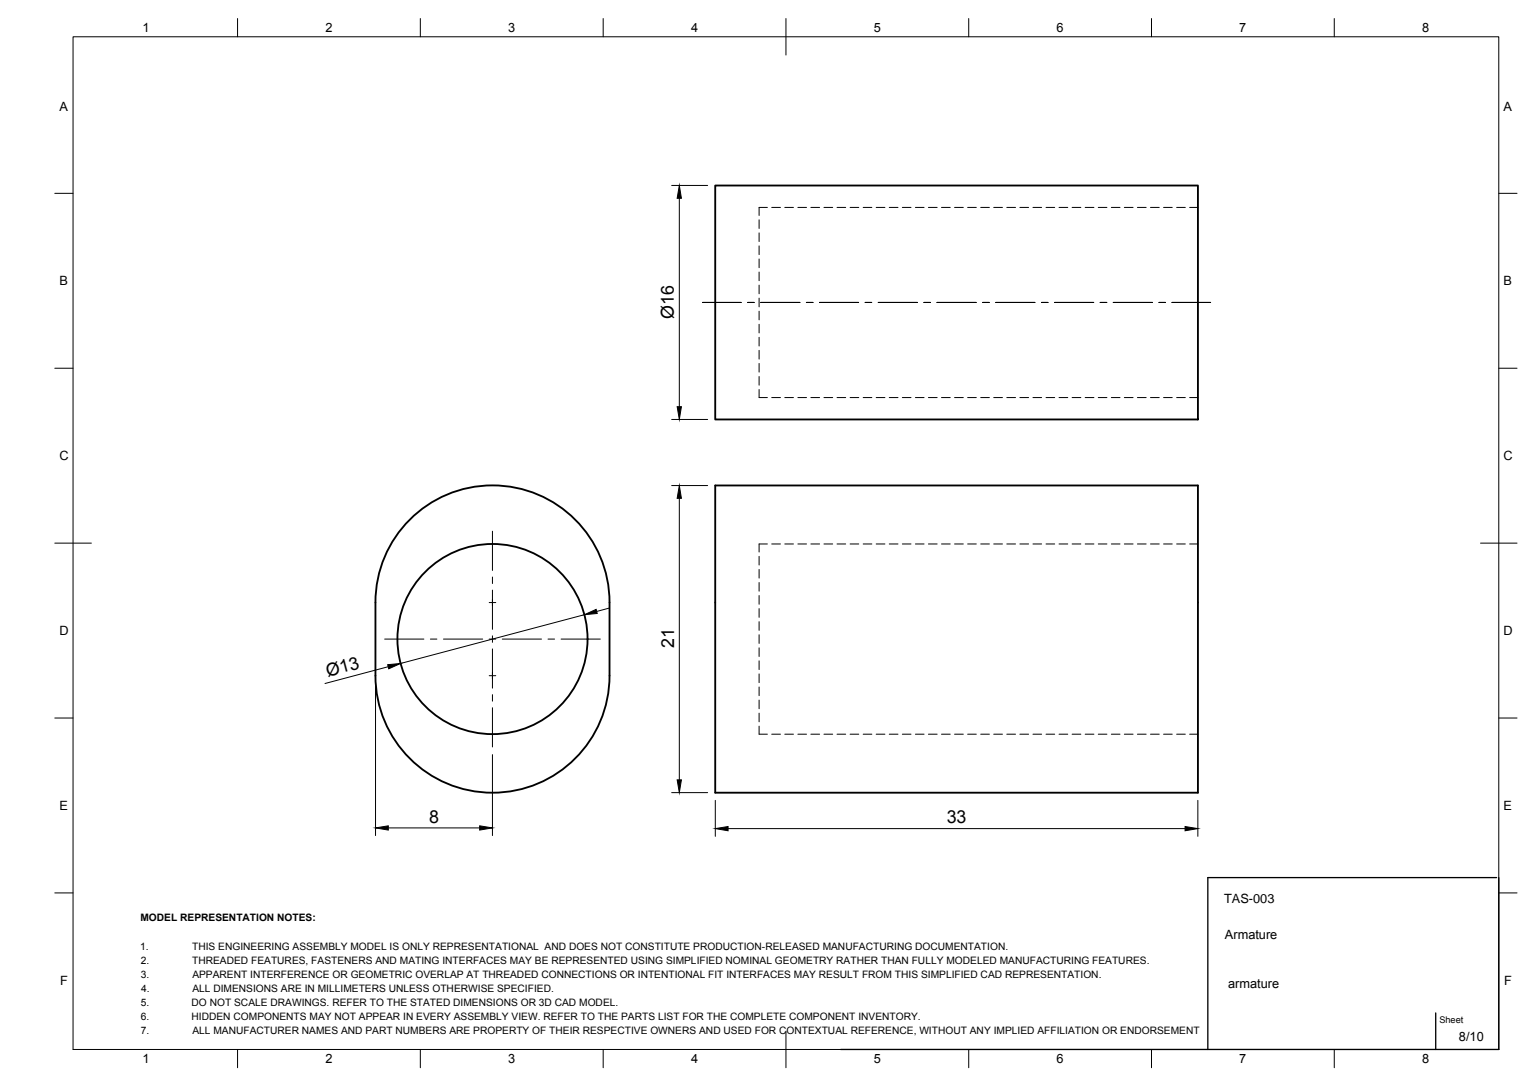
ISO-10303-21;
HEADER;
/* Generated by software containing ST-Developer
 * from STEP Tools, Inc. (www.steptools.com) 
 */

FILE_DESCRIPTION(
/* description */ ('STEP AP214'),
/* implementation_level */ '2;1');

FILE_NAME(
/* name */ 'armature.step',
/* time_stamp */ '2026-11-04T19:43:37-08:00',
/* author */ (''),
/* organization */ (''),
/* preprocessor_version */ 'ST-DEVELOPER v20.2',
/* originating_system */ 'Autodesk Translation Framework v15.17.0.0',
/* authorisation */ '');

FILE_SCHEMA (('AUTOMOTIVE_DESIGN { 1 0 10303 214 3 1 1 }'));
ENDSEC;

DATA;
#10=MECHANICAL_DESIGN_GEOMETRIC_PRESENTATION_REPRESENTATION('',(#120),#7627);
#102=SHAPE_REPRESENTATION_RELATIONSHIP('SRR','None',#7670,#111);
#111=ADVANCED_BREP_SHAPE_REPRESENTATION('',(#141),#7623);
#120=STYLED_ITEM('',(#7723),#141);
#141=MANIFOLD_SOLID_BREP('Body1',#2418);
#178=FACE_BOUND('',#536,.T.);
#217=PLANE('',#2637);
#218=PLANE('',#2641);
#219=PLANE('',#2642);
#220=PLANE('',#2643);
#221=PLANE('',#2644);
#273=CYLINDRICAL_SURFACE('',#2631,6.5);
#274=CYLINDRICAL_SURFACE('',#2634,8.);
#275=CYLINDRICAL_SURFACE('',#2639,8.);
#358=FACE_OUTER_BOUND('',#533,.T.);
#359=FACE_OUTER_BOUND('',#534,.T.);
#360=FACE_OUTER_BOUND('',#535,.T.);
#361=FACE_OUTER_BOUND('',#537,.T.);
#362=FACE_OUTER_BOUND('',#538,.T.);
#363=FACE_OUTER_BOUND('',#539,.T.);
#364=FACE_OUTER_BOUND('',#540,.T.);
#365=FACE_OUTER_BOUND('',#541,.T.);
#533=EDGE_LOOP('',(#1819,#1820,#1821,#1822));
#534=EDGE_LOOP('',(#1823,#1824,#1825,#1826));
#535=EDGE_LOOP('',(#1827,#1828,#1829,#1830));
#536=EDGE_LOOP('',(#1831));
#537=EDGE_LOOP('',(#1832,#1833,#1834,#1835));
#538=EDGE_LOOP('',(#1836,#1837,#1838,#1839));
#539=EDGE_LOOP('',(#1840,#1841,#1842,#1843));
#540=EDGE_LOOP('',(#1844));
#541=EDGE_LOOP('',(#1845,#1846,#1847,#1848));
#689=CIRCLE('',#2632,6.5);
#690=CIRCLE('',#2633,6.5);
#691=CIRCLE('',#2635,8.);
#692=CIRCLE('',#2636,8.);
#693=CIRCLE('',#2638,8.);
#694=CIRCLE('',#2640,8.);
#856=LINE('',#7150,#1012);
#857=LINE('',#7157,#1013);
#858=LINE('',#7160,#1014);
#859=LINE('',#7165,#1015);
#860=LINE('',#7166,#1016);
#861=LINE('',#7169,#1017);
#862=LINE('',#7172,#1018);
#863=LINE('',#7174,#1019);
#864=LINE('',#7176,#1020);
#1012=VECTOR('',#3115,6.5);
#1013=VECTOR('',#3122,1000.);
#1014=VECTOR('',#3125,1000.);
#1015=VECTOR('',#3130,1000.);
#1016=VECTOR('',#3131,1000.);
#1017=VECTOR('',#3134,1000.);
#1018=VECTOR('',#3137,1000.);
#1019=VECTOR('',#3140,1000.);
#1020=VECTOR('',#3143,1000.);
#1181=VERTEX_POINT('',#7147);
#1182=VERTEX_POINT('',#7149);
#1183=VERTEX_POINT('',#7153);
#1184=VERTEX_POINT('',#7154);
#1185=VERTEX_POINT('',#7156);
#1186=VERTEX_POINT('',#7158);
#1187=VERTEX_POINT('',#7162);
#1188=VERTEX_POINT('',#7163);
#1189=VERTEX_POINT('',#7168);
#1190=VERTEX_POINT('',#7170);
#1404=EDGE_CURVE('',#1181,#1181,#689,.T.);
#1405=EDGE_CURVE('',#1181,#1182,#856,.T.);
#1406=EDGE_CURVE('',#1182,#1182,#690,.T.);
#1407=EDGE_CURVE('',#1183,#1184,#691,.T.);
#1408=EDGE_CURVE('',#1183,#1185,#857,.T.);
#1409=EDGE_CURVE('',#1185,#1186,#692,.T.);
#1410=EDGE_CURVE('',#1184,#1186,#858,.T.);
#1411=EDGE_CURVE('',#1187,#1188,#693,.T.);
#1412=EDGE_CURVE('',#1186,#1187,#859,.T.);
#1413=EDGE_CURVE('',#1188,#1185,#860,.T.);
#1414=EDGE_CURVE('',#1189,#1188,#861,.T.);
#1415=EDGE_CURVE('',#1190,#1189,#694,.T.);
#1416=EDGE_CURVE('',#1190,#1187,#862,.T.);
#1417=EDGE_CURVE('',#1189,#1183,#863,.T.);
#1418=EDGE_CURVE('',#1184,#1190,#864,.T.);
#1819=ORIENTED_EDGE('',*,*,#1404,.T.);
#1820=ORIENTED_EDGE('',*,*,#1405,.T.);
#1821=ORIENTED_EDGE('',*,*,#1406,.F.);
#1822=ORIENTED_EDGE('',*,*,#1405,.F.);
#1823=ORIENTED_EDGE('',*,*,#1407,.F.);
#1824=ORIENTED_EDGE('',*,*,#1408,.T.);
#1825=ORIENTED_EDGE('',*,*,#1409,.T.);
#1826=ORIENTED_EDGE('',*,*,#1410,.F.);
#1827=ORIENTED_EDGE('',*,*,#1411,.F.);
#1828=ORIENTED_EDGE('',*,*,#1412,.F.);
#1829=ORIENTED_EDGE('',*,*,#1409,.F.);
#1830=ORIENTED_EDGE('',*,*,#1413,.F.);
#1831=ORIENTED_EDGE('',*,*,#1406,.T.);
#1832=ORIENTED_EDGE('',*,*,#1411,.T.);
#1833=ORIENTED_EDGE('',*,*,#1414,.F.);
#1834=ORIENTED_EDGE('',*,*,#1415,.F.);
#1835=ORIENTED_EDGE('',*,*,#1416,.T.);
#1836=ORIENTED_EDGE('',*,*,#1413,.T.);
#1837=ORIENTED_EDGE('',*,*,#1408,.F.);
#1838=ORIENTED_EDGE('',*,*,#1417,.F.);
#1839=ORIENTED_EDGE('',*,*,#1414,.T.);
#1840=ORIENTED_EDGE('',*,*,#1412,.T.);
#1841=ORIENTED_EDGE('',*,*,#1416,.F.);
#1842=ORIENTED_EDGE('',*,*,#1418,.F.);
#1843=ORIENTED_EDGE('',*,*,#1410,.T.);
#1844=ORIENTED_EDGE('',*,*,#1404,.F.);
#1845=ORIENTED_EDGE('',*,*,#1415,.T.);
#1846=ORIENTED_EDGE('',*,*,#1417,.T.);
#1847=ORIENTED_EDGE('',*,*,#1407,.T.);
#1848=ORIENTED_EDGE('',*,*,#1418,.T.);
#2309=ADVANCED_FACE('',(#358),#273,.F.);
#2310=ADVANCED_FACE('',(#359),#274,.T.);
#2311=ADVANCED_FACE('',(#360,#178),#217,.F.);
#2312=ADVANCED_FACE('',(#361),#275,.T.);
#2313=ADVANCED_FACE('',(#362),#218,.F.);
#2314=ADVANCED_FACE('',(#363),#219,.F.);
#2315=ADVANCED_FACE('',(#364),#220,.F.);
#2316=ADVANCED_FACE('',(#365),#221,.T.);
#2418=CLOSED_SHELL('',(#2309,#2310,#2311,#2312,#2313,#2314,#2315,#2316));
#2630=AXIS2_PLACEMENT_3D('',#7145,#3109,#3110);
#2631=AXIS2_PLACEMENT_3D('',#7146,#3111,#3112);
#2632=AXIS2_PLACEMENT_3D('',#7148,#3113,#3114);
#2633=AXIS2_PLACEMENT_3D('',#7151,#3116,#3117);
#2634=AXIS2_PLACEMENT_3D('',#7152,#3118,#3119);
#2635=AXIS2_PLACEMENT_3D('',#7155,#3120,#3121);
#2636=AXIS2_PLACEMENT_3D('',#7159,#3123,#3124);
#2637=AXIS2_PLACEMENT_3D('',#7161,#3126,#3127);
#2638=AXIS2_PLACEMENT_3D('',#7164,#3128,#3129);
#2639=AXIS2_PLACEMENT_3D('',#7167,#3132,#3133);
#2640=AXIS2_PLACEMENT_3D('',#7171,#3135,#3136);
#2641=AXIS2_PLACEMENT_3D('',#7173,#3138,#3139);
#2642=AXIS2_PLACEMENT_3D('',#7175,#3141,#3142);
#2643=AXIS2_PLACEMENT_3D('',#7177,#3144,#3145);
#2644=AXIS2_PLACEMENT_3D('',#7178,#3146,#3147);
#3109=DIRECTION('axis',(0.,0.,1.));
#3110=DIRECTION('refdir',(1.,0.,0.));
#3111=DIRECTION('center_axis',(0.,-1.,0.));
#3112=DIRECTION('ref_axis',(0.,0.,-1.));
#3113=DIRECTION('center_axis',(0.,1.,0.));
#3114=DIRECTION('ref_axis',(0.,0.,1.));
#3115=DIRECTION('',(0.,-1.,0.));
#3116=DIRECTION('center_axis',(0.,1.,0.));
#3117=DIRECTION('ref_axis',(0.,0.,1.));
#3118=DIRECTION('center_axis',(0.,-1.,0.));
#3119=DIRECTION('ref_axis',(0.,0.,-1.));
#3120=DIRECTION('center_axis',(0.,1.,0.));
#3121=DIRECTION('ref_axis',(0.,0.,1.));
#3122=DIRECTION('',(0.,-1.,0.));
#3123=DIRECTION('center_axis',(0.,1.,0.));
#3124=DIRECTION('ref_axis',(0.,0.,1.));
#3125=DIRECTION('',(0.,-1.,0.));
#3126=DIRECTION('center_axis',(0.,1.,0.));
#3127=DIRECTION('ref_axis',(0.,0.,1.));
#3128=DIRECTION('center_axis',(0.,1.,0.));
#3129=DIRECTION('ref_axis',(0.,0.,1.));
#3130=DIRECTION('',(3.46944695195362E-16,0.,1.));
#3131=DIRECTION('',(-3.46944695195361E-16,0.,-1.));
#3132=DIRECTION('center_axis',(0.,-1.,0.));
#3133=DIRECTION('ref_axis',(1.22464679914735E-16,0.,1.));
#3134=DIRECTION('',(0.,-1.,0.));
#3135=DIRECTION('center_axis',(0.,1.,0.));
#3136=DIRECTION('ref_axis',(0.,0.,1.));
#3137=DIRECTION('',(0.,-1.,0.));
#3138=DIRECTION('center_axis',(-1.,0.,3.46944695195361E-16));
#3139=DIRECTION('ref_axis',(3.46944695195361E-16,0.,1.));
#3140=DIRECTION('',(-3.46944695195361E-16,0.,-1.));
#3141=DIRECTION('center_axis',(1.,0.,-3.46944695195362E-16));
#3142=DIRECTION('ref_axis',(-3.46944695195362E-16,0.,-1.));
#3143=DIRECTION('',(3.46944695195361E-16,0.,1.));
#3144=DIRECTION('center_axis',(0.,1.,0.));
#3145=DIRECTION('ref_axis',(0.,0.,1.));
#3146=DIRECTION('center_axis',(0.,1.,0.));
#3147=DIRECTION('ref_axis',(0.,0.,1.));
#7145=CARTESIAN_POINT('',(0.,0.,0.));
#7146=CARTESIAN_POINT('Origin',(0.,43.,0.));
#7147=CARTESIAN_POINT('',(-7.96020419445779E-16,43.,6.5));
#7148=CARTESIAN_POINT('Origin',(0.,43.,0.));
#7149=CARTESIAN_POINT('',(-7.96020419445779E-16,13.,6.5));
#7150=CARTESIAN_POINT('',(-7.96020419445779E-16,43.,6.5));
#7151=CARTESIAN_POINT('Origin',(0.,13.,0.));
#7152=CARTESIAN_POINT('Origin',(-9.18485099360515E-16,43.,-2.5));
#7153=CARTESIAN_POINT('',(8.,46.,-2.5));
#7154=CARTESIAN_POINT('',(-8.,46.,-2.5));
#7155=CARTESIAN_POINT('Origin',(-9.18485099360515E-16,46.,-2.5));
#7156=CARTESIAN_POINT('',(8.,13.,-2.5));
#7157=CARTESIAN_POINT('',(8.,43.,-2.5));
#7158=CARTESIAN_POINT('',(-8.,13.,-2.5));
#7159=CARTESIAN_POINT('Origin',(-9.18485099360515E-16,13.,-2.5));
#7160=CARTESIAN_POINT('',(-8.,43.,-2.5));
#7161=CARTESIAN_POINT('Origin',(0.,13.,2.5));
#7162=CARTESIAN_POINT('',(-8.,13.,2.5));
#7163=CARTESIAN_POINT('',(8.,13.,2.5));
#7164=CARTESIAN_POINT('Origin',(0.,13.,2.5));
#7165=CARTESIAN_POINT('',(-8.,13.,2.5));
#7166=CARTESIAN_POINT('',(8.,13.,2.5));
#7167=CARTESIAN_POINT('Origin',(0.,43.,2.5));
#7168=CARTESIAN_POINT('',(8.,46.,2.5));
#7169=CARTESIAN_POINT('',(8.,43.,2.5));
#7170=CARTESIAN_POINT('',(-8.,46.,2.5));
#7171=CARTESIAN_POINT('Origin',(0.,46.,2.5));
#7172=CARTESIAN_POINT('',(-8.,43.,2.5));
#7173=CARTESIAN_POINT('Origin',(8.,43.,2.5));
#7174=CARTESIAN_POINT('',(8.,46.,2.5));
#7175=CARTESIAN_POINT('Origin',(-8.,43.,2.5));
#7176=CARTESIAN_POINT('',(-8.,46.,2.5));
#7177=CARTESIAN_POINT('Origin',(0.,43.,2.5));
#7178=CARTESIAN_POINT('Origin',(0.,46.,2.5));
#7612=UNCERTAINTY_MEASURE_WITH_UNIT(LENGTH_MEASURE(0.01),#7628,
'DISTANCE_ACCURACY_VALUE',
'Maximum model space distance between geometric entities at asserted c
onnectivities');
#7616=UNCERTAINTY_MEASURE_WITH_UNIT(LENGTH_MEASURE(0.01),#7628,
'DISTANCE_ACCURACY_VALUE',
'Maximum model space distance between geometric entities at asserted c
onnectivities');
#7623=(
GEOMETRIC_REPRESENTATION_CONTEXT(3)
GLOBAL_UNCERTAINTY_ASSIGNED_CONTEXT((#7612))
GLOBAL_UNIT_ASSIGNED_CONTEXT((#7628,#7630,#7631))
REPRESENTATION_CONTEXT('','3D')
);
#7627=(
GEOMETRIC_REPRESENTATION_CONTEXT(3)
GLOBAL_UNCERTAINTY_ASSIGNED_CONTEXT((#7616))
GLOBAL_UNIT_ASSIGNED_CONTEXT((#7628,#7630,#7631))
REPRESENTATION_CONTEXT('','3D')
);
#7628=(
LENGTH_UNIT()
NAMED_UNIT(*)
SI_UNIT(.MILLI.,.METRE.)
);
#7630=(
NAMED_UNIT(*)
PLANE_ANGLE_UNIT()
SI_UNIT($,.RADIAN.)
);
#7631=(
NAMED_UNIT(*)
SI_UNIT($,.STERADIAN.)
SOLID_ANGLE_UNIT()
);
#7638=SHAPE_DEFINITION_REPRESENTATION(#7648,#7670);
#7648=PRODUCT_DEFINITION_SHAPE('',$,#7681);
#7670=SHAPE_REPRESENTATION('',(#2630),#7623);
#7674=PRODUCT_DEFINITION_CONTEXT('part definition',#7706,'design');
#7681=PRODUCT_DEFINITION('armature','armature',#7691,#7674);
#7691=PRODUCT_DEFINITION_FORMATION('',$,#7714);
#7706=APPLICATION_CONTEXT(
'Core Data for Automotive Mechanical Design Process');
#7707=PRODUCT_CONTEXT('part definition',#7706,'mechanical');
#7714=PRODUCT('armature','armature',$,(#7707));
#7723=PRESENTATION_STYLE_ASSIGNMENT((#7729));
#7729=SURFACE_STYLE_USAGE(.BOTH.,#7735);
#7735=SURFACE_SIDE_STYLE('',(#7741));
#7741=SURFACE_STYLE_FILL_AREA(#7747);
#7747=FILL_AREA_STYLE('Opaque(97,158,199)',(#7753));
#7753=FILL_AREA_STYLE_COLOUR('Opaque(97,158,199)',#7759);
#7759=COLOUR_RGB('Opaque(97,158,199)',0.380392156862745,0.619607843137255,
0.780392156862745);
ENDSEC;
END-ISO-10303-21;
